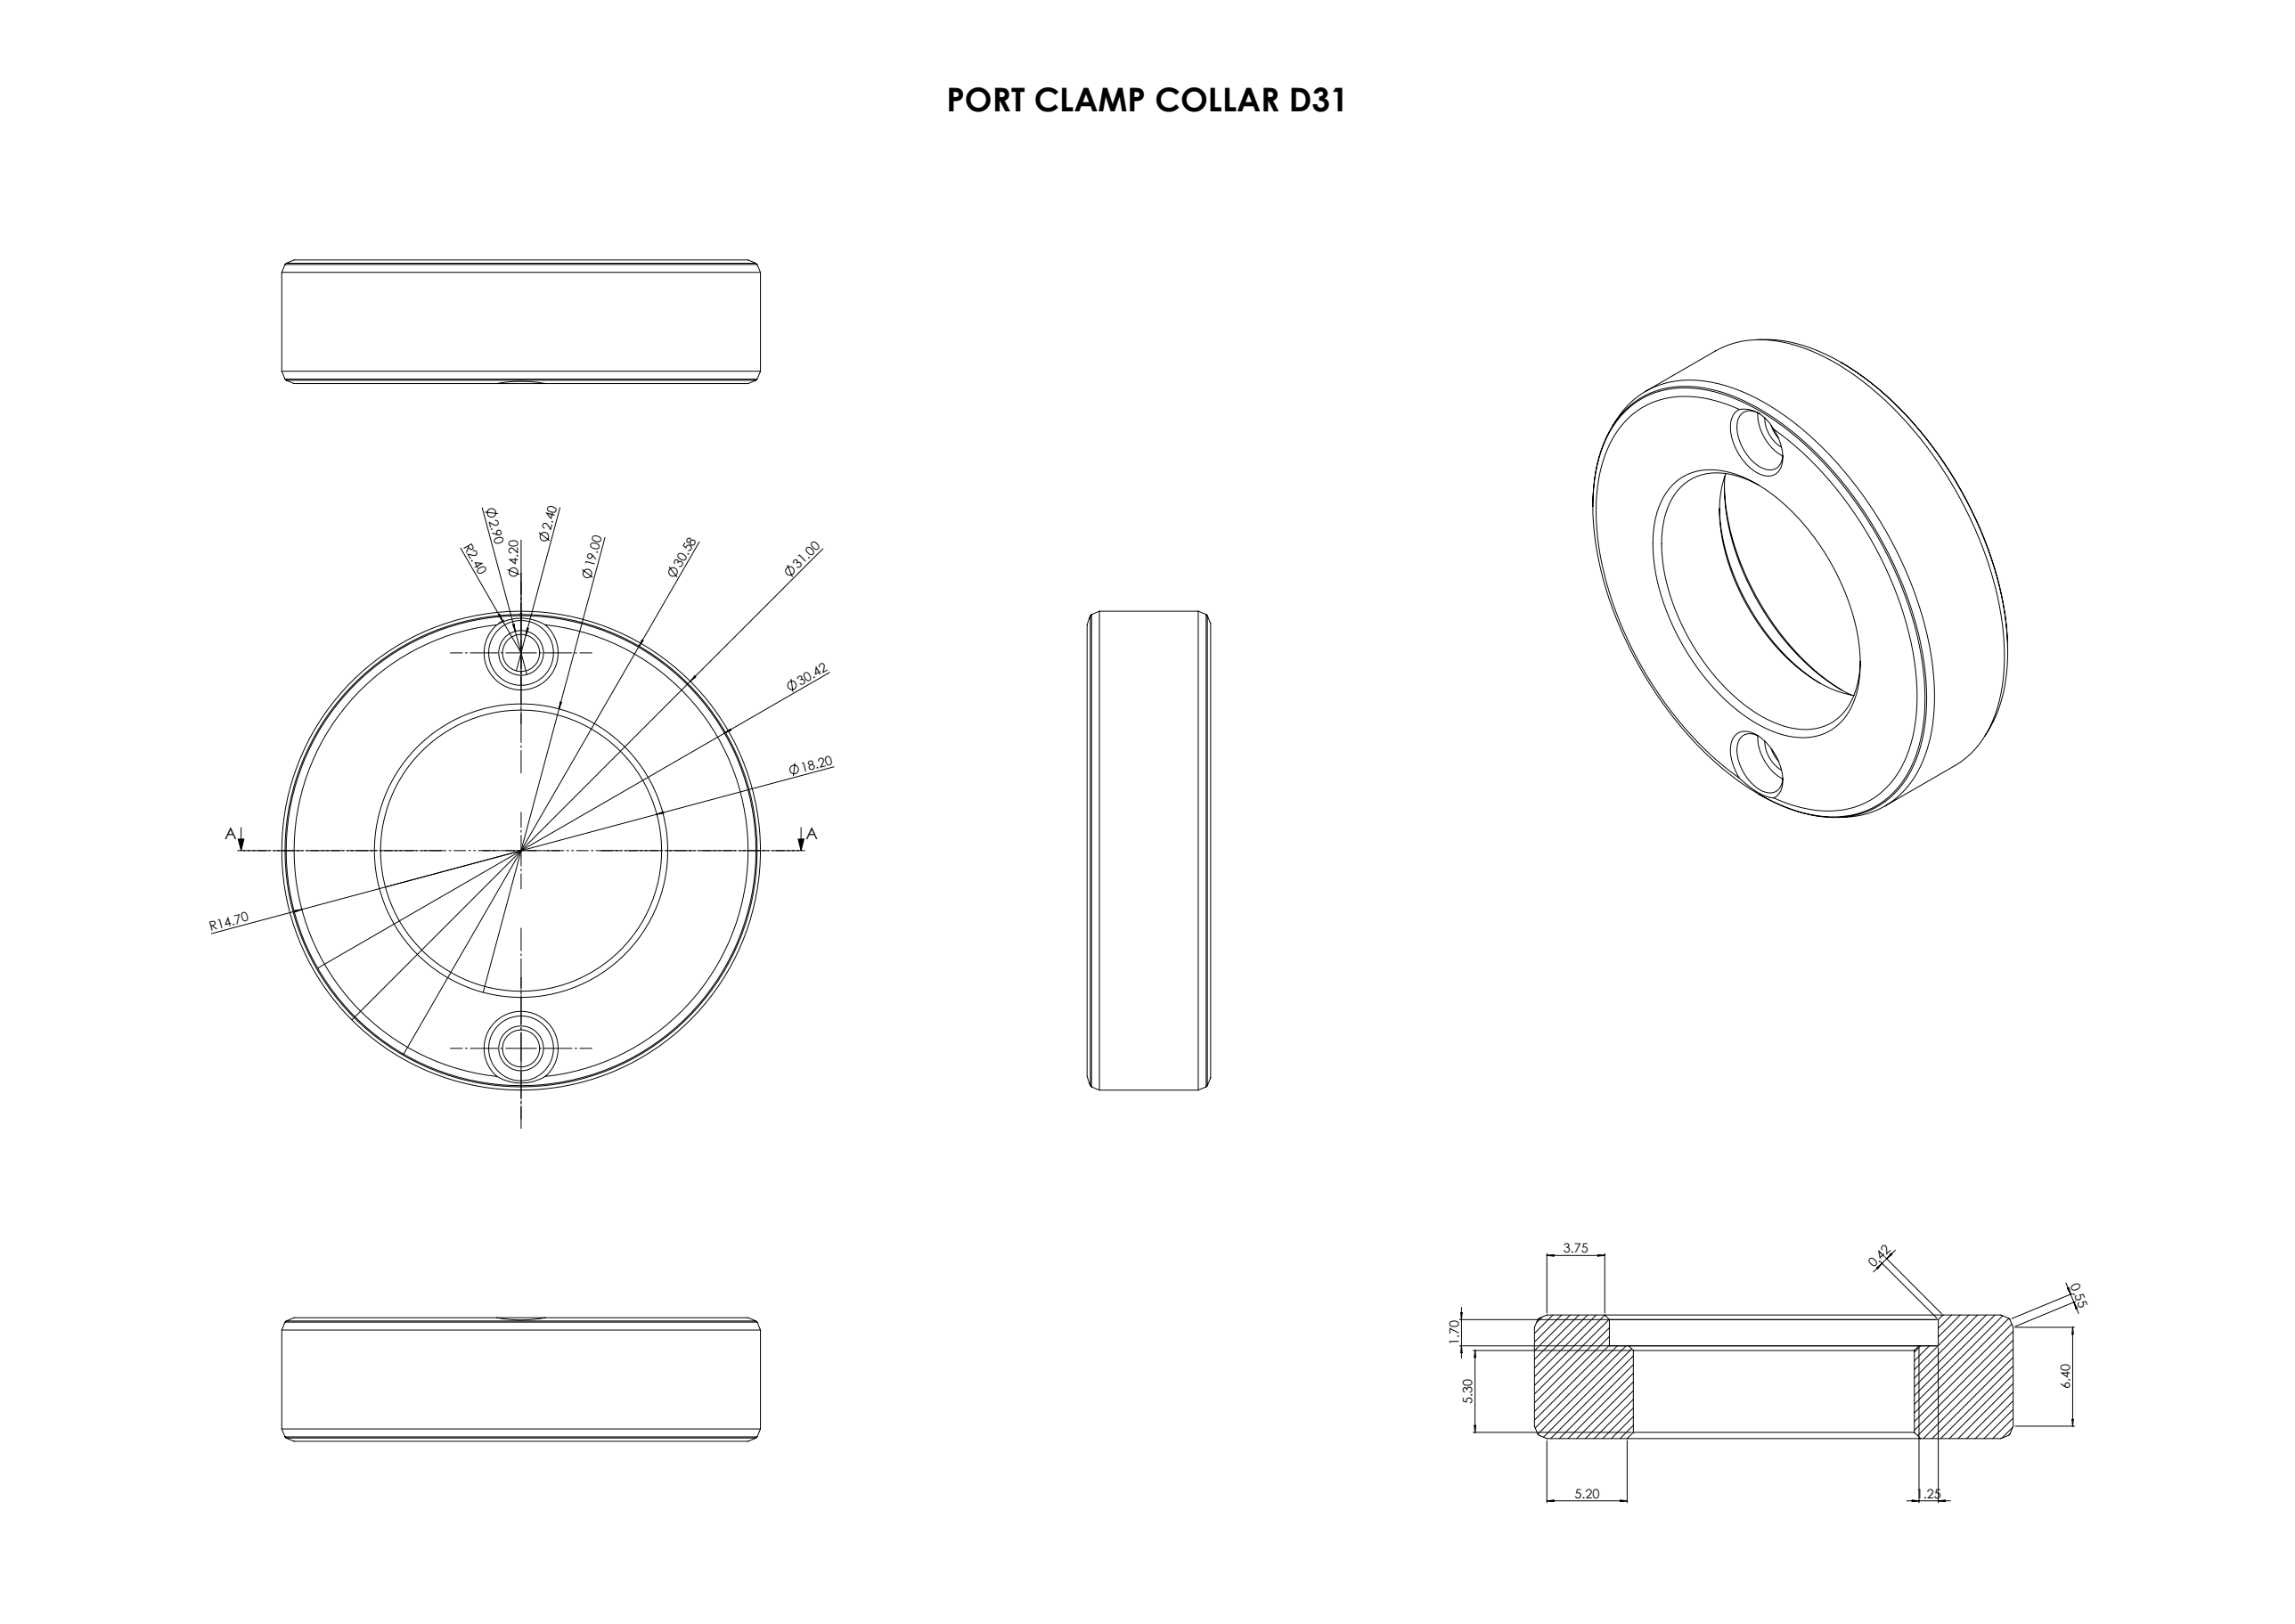
ISO-10303-21;
HEADER;
/* Generated by software containing ST-Developer
 * from STEP Tools, Inc. (www.steptools.com) 
 */

FILE_DESCRIPTION(
/* description */ (''),
/* implementation_level */ '2;1');

FILE_NAME(
/* name */ '05_Port_Clamp_Collar_D31.step',
/* time_stamp */ '2026-10-19T23:00:43-07:00',
/* author */ (''),
/* organization */ (''),
/* preprocessor_version */ 'ST-DEVELOPER v20.2',
/* originating_system */ 'Autodesk Translation Framework v15.15.0.0',
/* authorisation */ '');

FILE_SCHEMA (('AUTOMOTIVE_DESIGN { 1 0 10303 214 3 1 1 }'));
ENDSEC;

DATA;
#10=MECHANICAL_DESIGN_GEOMETRIC_PRESENTATION_REPRESENTATION('',(#1000),#55002);
#484=B_SPLINE_CURVE_WITH_KNOTS('',3,(#36025,#36026,#36027,#36028,#36029,
#36030,#36031,#36032,#36033,#36034),.UNSPECIFIED.,.F.,.F.,(4,2,2,2,4),(0.529829601296569,
0.55431923537737,0.690027699159176,0.825736162940983,0.850225797021783),
 .UNSPECIFIED.);
#485=B_SPLINE_CURVE_WITH_KNOTS('',3,(#36038,#36039,#36040,#36041,#36042,
#36043,#36044,#36045,#36046,#36047),.UNSPECIFIED.,.F.,.F.,(4,2,2,2,4),(0.529829601296585,
0.554319235377384,0.690027699159196,0.825736162941008,0.850225797021807),
 .UNSPECIFIED.);
#960=SHAPE_REPRESENTATION_RELATIONSHIP('SRR','None',#55108,#980);
#980=ADVANCED_BREP_SHAPE_REPRESENTATION('',(#1020),#54986);
#1000=STYLED_ITEM('',(#55379),#1020);
#1020=MANIFOLD_SOLID_BREP('Port Clamp Collar',#24533);
#1162=FACE_BOUND('',#4344,.T.);
#1163=FACE_BOUND('',#4345,.T.);
#1164=FACE_BOUND('',#4346,.T.);
#1165=FACE_BOUND('',#4357,.T.);
#1166=FACE_BOUND('',#4367,.T.);
#1167=FACE_BOUND('',#4372,.T.);
#1168=FACE_BOUND('',#4375,.T.);
#1418=PLANE('',#25686);
#1419=PLANE('',#25713);
#1420=PLANE('',#25738);
#1421=PLANE('',#25745);
#1422=PLANE('',#25748);
#2121=CYLINDRICAL_SURFACE('',#25690,1.065);
#2122=CYLINDRICAL_SURFACE('',#25699,1.55);
#2123=CYLINDRICAL_SURFACE('',#25710,0.91);
#2124=CYLINDRICAL_SURFACE('',#25723,0.21);
#2125=CYLINDRICAL_SURFACE('',#25730,0.21);
#2126=CYLINDRICAL_SURFACE('',#25734,0.12);
#2127=CYLINDRICAL_SURFACE('',#25741,0.12);
#2852=FACE_OUTER_BOUND('',#4342,.T.);
#2853=FACE_OUTER_BOUND('',#4343,.T.);
#2854=FACE_OUTER_BOUND('',#4347,.T.);
#2855=FACE_OUTER_BOUND('',#4348,.T.);
#2856=FACE_OUTER_BOUND('',#4349,.T.);
#2857=FACE_OUTER_BOUND('',#4350,.T.);
#2858=FACE_OUTER_BOUND('',#4351,.T.);
#2859=FACE_OUTER_BOUND('',#4352,.T.);
#2860=FACE_OUTER_BOUND('',#4353,.T.);
#2861=FACE_OUTER_BOUND('',#4354,.T.);
#2862=FACE_OUTER_BOUND('',#4355,.T.);
#2863=FACE_OUTER_BOUND('',#4356,.T.);
#2864=FACE_OUTER_BOUND('',#4358,.T.);
#2865=FACE_OUTER_BOUND('',#4359,.T.);
#2866=FACE_OUTER_BOUND('',#4360,.T.);
#2867=FACE_OUTER_BOUND('',#4361,.T.);
#2868=FACE_OUTER_BOUND('',#4362,.T.);
#2869=FACE_OUTER_BOUND('',#4363,.T.);
#2870=FACE_OUTER_BOUND('',#4364,.T.);
#2871=FACE_OUTER_BOUND('',#4365,.T.);
#2872=FACE_OUTER_BOUND('',#4366,.T.);
#2873=FACE_OUTER_BOUND('',#4368,.T.);
#2874=FACE_OUTER_BOUND('',#4369,.T.);
#2875=FACE_OUTER_BOUND('',#4370,.T.);
#2876=FACE_OUTER_BOUND('',#4371,.T.);
#2877=FACE_OUTER_BOUND('',#4373,.T.);
#2878=FACE_OUTER_BOUND('',#4374,.T.);
#4342=EDGE_LOOP('',(#17878,#17879,#17880,#17881,#17882));
#4343=EDGE_LOOP('',(#17883));
#4344=EDGE_LOOP('',(#17884));
#4345=EDGE_LOOP('',(#17885));
#4346=EDGE_LOOP('',(#17886));
#4347=EDGE_LOOP('',(#17887,#17888,#17889,#17890,#17891));
#4348=EDGE_LOOP('',(#17892,#17893,#17894,#17895));
#4349=EDGE_LOOP('',(#17896,#17897,#17898,#17899));
#4350=EDGE_LOOP('',(#17900,#17901,#17902,#17903,#17904));
#4351=EDGE_LOOP('',(#17905,#17906,#17907,#17908,#17909,#17910));
#4352=EDGE_LOOP('',(#17911,#17912,#17913,#17914,#17915));
#4353=EDGE_LOOP('',(#17916,#17917,#17918,#17919));
#4354=EDGE_LOOP('',(#17920,#17921,#17922,#17923,#17924));
#4355=EDGE_LOOP('',(#17925,#17926,#17927,#17928,#17929,#17930));
#4356=EDGE_LOOP('',(#17931));
#4357=EDGE_LOOP('',(#17932));
#4358=EDGE_LOOP('',(#17933,#17934,#17935,#17936,#17937,#17938,#17939,#17940));
#4359=EDGE_LOOP('',(#17941,#17942,#17943,#17944,#17945,#17946,#17947));
#4360=EDGE_LOOP('',(#17948,#17949,#17950,#17951,#17952));
#4361=EDGE_LOOP('',(#17953,#17954,#17955,#17956,#17957,#17958,#17959));
#4362=EDGE_LOOP('',(#17960,#17961,#17962,#17963,#17964));
#4363=EDGE_LOOP('',(#17965,#17966,#17967,#17968));
#4364=EDGE_LOOP('',(#17969,#17970,#17971,#17972));
#4365=EDGE_LOOP('',(#17973,#17974,#17975,#17976));
#4366=EDGE_LOOP('',(#17977));
#4367=EDGE_LOOP('',(#17978));
#4368=EDGE_LOOP('',(#17979,#17980,#17981,#17982));
#4369=EDGE_LOOP('',(#17983,#17984,#17985,#17986));
#4370=EDGE_LOOP('',(#17987,#17988,#17989,#17990));
#4371=EDGE_LOOP('',(#17991));
#4372=EDGE_LOOP('',(#17992));
#4373=EDGE_LOOP('',(#17993,#17994,#17995,#17996,#17997));
#4374=EDGE_LOOP('',(#17998,#17999,#18000,#18001,#18002,#18003,#18004));
#4375=EDGE_LOOP('',(#18005));
#5910=LINE('',#35961,#7731);
#5911=LINE('',#35975,#7732);
#5912=LINE('',#35979,#7733);
#5913=LINE('',#35983,#7734);
#5914=LINE('',#35986,#7735);
#5915=LINE('',#35995,#7736);
#5916=LINE('',#35999,#7737);
#5917=LINE('',#36003,#7738);
#5918=LINE('',#36008,#7739);
#5919=LINE('',#36017,#7740);
#5920=LINE('',#36021,#7741);
#5921=LINE('',#36053,#7742);
#5922=LINE('',#36061,#7743);
#5923=LINE('',#36066,#7744);
#5924=LINE('',#36074,#7745);
#5925=LINE('',#36077,#7746);
#5926=LINE('',#36081,#7747);
#5927=LINE('',#36085,#7748);
#5928=LINE('',#36090,#7749);
#5929=LINE('',#36094,#7750);
#5930=LINE('',#36098,#7751);
#5931=LINE('',#36103,#7752);
#7731=VECTOR('',#29554,1.08);
#7732=VECTOR('',#29571,1.065);
#7733=VECTOR('',#29576,1.4956066017178);
#7734=VECTOR('',#29581,1.525);
#7735=VECTOR('',#29584,1.5393933982822);
#7736=VECTOR('',#29595,1.55);
#7737=VECTOR('',#29600,1.5393933982822);
#7738=VECTOR('',#29605,1.525);
#7739=VECTOR('',#29610,0.925);
#7740=VECTOR('',#29621,0.91);
#7741=VECTOR('',#29626,1.4956066017178);
#7742=VECTOR('',#29637,0.225);
#7743=VECTOR('',#29648,0.21);
#7744=VECTOR('',#29653,0.225);
#7745=VECTOR('',#29664,0.21);
#7746=VECTOR('',#29667,0.1325);
#7747=VECTOR('',#29672,0.12);
#7748=VECTOR('',#29677,0.1325);
#7749=VECTOR('',#29684,0.1325);
#7750=VECTOR('',#29689,0.12);
#7751=VECTOR('',#29694,0.1325);
#7752=VECTOR('',#29701,0.93);
#9488=CIRCLE('',#25683,1.095);
#9489=CIRCLE('',#25684,1.065);
#9490=CIRCLE('',#25685,1.065);
#9491=CIRCLE('',#25687,1.47);
#9492=CIRCLE('',#25688,0.128333333333334);
#9493=CIRCLE('',#25689,0.128333333333334);
#9494=CIRCLE('',#25691,1.065);
#9495=CIRCLE('',#25693,1.5212132034356);
#9496=CIRCLE('',#25695,1.5287867965644);
#9497=CIRCLE('',#25697,1.55);
#9498=CIRCLE('',#25698,1.55);
#9499=CIRCLE('',#25700,1.55);
#9500=CIRCLE('',#25701,1.55);
#9501=CIRCLE('',#25703,1.5287867965644);
#9502=CIRCLE('',#25705,1.5212132034356);
#9503=CIRCLE('',#25707,0.94);
#9504=CIRCLE('',#25708,0.91);
#9505=CIRCLE('',#25709,0.91);
#9506=CIRCLE('',#25711,0.91);
#9507=CIRCLE('',#25712,0.91);
#9508=CIRCLE('',#25715,1.47);
#9509=CIRCLE('',#25716,1.47);
#9510=CIRCLE('',#25717,1.47);
#9511=CIRCLE('',#25719,0.24);
#9512=CIRCLE('',#25720,0.21);
#9513=CIRCLE('',#25721,0.21);
#9514=CIRCLE('',#25722,0.24);
#9515=CIRCLE('',#25724,0.21);
#9516=CIRCLE('',#25726,0.24);
#9517=CIRCLE('',#25727,0.21);
#9518=CIRCLE('',#25728,0.21);
#9519=CIRCLE('',#25729,0.24);
#9520=CIRCLE('',#25731,0.21);
#9521=CIRCLE('',#25733,0.12);
#9522=CIRCLE('',#25735,0.12);
#9523=CIRCLE('',#25737,0.145);
#9524=CIRCLE('',#25740,0.12);
#9525=CIRCLE('',#25742,0.12);
#9526=CIRCLE('',#25744,0.145);
#9527=CIRCLE('',#25747,0.95);
#10672=VERTEX_POINT('',#35958);
#10673=VERTEX_POINT('',#35960);
#10674=VERTEX_POINT('',#35962);
#10675=VERTEX_POINT('',#35966);
#10676=VERTEX_POINT('',#35968);
#10677=VERTEX_POINT('',#35970);
#10678=VERTEX_POINT('',#35973);
#10679=VERTEX_POINT('',#35977);
#10680=VERTEX_POINT('',#35981);
#10681=VERTEX_POINT('',#35985);
#10682=VERTEX_POINT('',#35987);
#10683=VERTEX_POINT('',#35991);
#10684=VERTEX_POINT('',#35992);
#10685=VERTEX_POINT('',#35997);
#10686=VERTEX_POINT('',#36001);
#10687=VERTEX_POINT('',#36005);
#10688=VERTEX_POINT('',#36007);
#10689=VERTEX_POINT('',#36009);
#10690=VERTEX_POINT('',#36013);
#10691=VERTEX_POINT('',#36014);
#10692=VERTEX_POINT('',#36020);
#10693=VERTEX_POINT('',#36022);
#10694=VERTEX_POINT('',#36024);
#10695=VERTEX_POINT('',#36035);
#10696=VERTEX_POINT('',#36037);
#10697=VERTEX_POINT('',#36050);
#10698=VERTEX_POINT('',#36052);
#10699=VERTEX_POINT('',#36054);
#10700=VERTEX_POINT('',#36059);
#10701=VERTEX_POINT('',#36063);
#10702=VERTEX_POINT('',#36065);
#10703=VERTEX_POINT('',#36067);
#10704=VERTEX_POINT('',#36072);
#10705=VERTEX_POINT('',#36076);
#10706=VERTEX_POINT('',#36080);
#10707=VERTEX_POINT('',#36084);
#10708=VERTEX_POINT('',#36089);
#10709=VERTEX_POINT('',#36093);
#10710=VERTEX_POINT('',#36097);
#10711=VERTEX_POINT('',#36102);
#13347=EDGE_CURVE('',#10672,#10672,#9488,.T.);
#13348=EDGE_CURVE('',#10672,#10673,#5910,.T.);
#13349=EDGE_CURVE('',#10673,#10674,#9489,.T.);
#13350=EDGE_CURVE('',#10674,#10673,#9490,.T.);
#13351=EDGE_CURVE('',#10675,#10675,#9491,.T.);
#13352=EDGE_CURVE('',#10676,#10676,#9492,.T.);
#13353=EDGE_CURVE('',#10677,#10677,#9493,.T.);
#13354=EDGE_CURVE('',#10678,#10678,#9494,.T.);
#13355=EDGE_CURVE('',#10678,#10674,#5911,.T.);
#13356=EDGE_CURVE('',#10679,#10679,#9495,.T.);
#13357=EDGE_CURVE('',#10679,#10675,#5912,.T.);
#13358=EDGE_CURVE('',#10680,#10680,#9496,.T.);
#13359=EDGE_CURVE('',#10680,#10679,#5913,.T.);
#13360=EDGE_CURVE('',#10680,#10681,#5914,.T.);
#13361=EDGE_CURVE('',#10681,#10682,#9497,.T.);
#13362=EDGE_CURVE('',#10682,#10681,#9498,.T.);
#13363=EDGE_CURVE('',#10683,#10684,#9499,.T.);
#13364=EDGE_CURVE('',#10684,#10683,#9500,.T.);
#13365=EDGE_CURVE('',#10684,#10682,#5915,.T.);
#13366=EDGE_CURVE('',#10685,#10685,#9501,.T.);
#13367=EDGE_CURVE('',#10685,#10683,#5916,.T.);
#13368=EDGE_CURVE('',#10686,#10686,#9502,.T.);
#13369=EDGE_CURVE('',#10686,#10685,#5917,.T.);
#13370=EDGE_CURVE('',#10687,#10687,#9503,.T.);
#13371=EDGE_CURVE('',#10687,#10688,#5918,.T.);
#13372=EDGE_CURVE('',#10688,#10689,#9504,.T.);
#13373=EDGE_CURVE('',#10689,#10688,#9505,.T.);
#13374=EDGE_CURVE('',#10690,#10691,#9506,.T.);
#13375=EDGE_CURVE('',#10691,#10690,#9507,.T.);
#13376=EDGE_CURVE('',#10691,#10689,#5919,.T.);
#13377=EDGE_CURVE('',#10686,#10692,#5920,.T.);
#13378=EDGE_CURVE('',#10692,#10693,#9508,.T.);
#13379=EDGE_CURVE('',#10694,#10693,#484,.T.);
#13380=EDGE_CURVE('',#10694,#10695,#9509,.T.);
#13381=EDGE_CURVE('',#10696,#10695,#485,.T.);
#13382=EDGE_CURVE('',#10696,#10692,#9510,.T.);
#13383=EDGE_CURVE('',#10695,#10697,#9511,.T.);
#13384=EDGE_CURVE('',#10697,#10698,#5921,.T.);
#13385=EDGE_CURVE('',#10698,#10699,#9512,.T.);
#13386=EDGE_CURVE('',#10699,#10698,#9513,.T.);
#13387=EDGE_CURVE('',#10697,#10696,#9514,.T.);
#13388=EDGE_CURVE('',#10700,#10700,#9515,.T.);
#13389=EDGE_CURVE('',#10700,#10699,#5922,.T.);
#13390=EDGE_CURVE('',#10693,#10701,#9516,.T.);
#13391=EDGE_CURVE('',#10701,#10702,#5923,.T.);
#13392=EDGE_CURVE('',#10702,#10703,#9517,.T.);
#13393=EDGE_CURVE('',#10703,#10702,#9518,.T.);
#13394=EDGE_CURVE('',#10701,#10694,#9519,.T.);
#13395=EDGE_CURVE('',#10704,#10704,#9520,.T.);
#13396=EDGE_CURVE('',#10704,#10703,#5924,.T.);
#13397=EDGE_CURVE('',#10676,#10705,#5925,.T.);
#13398=EDGE_CURVE('',#10705,#10705,#9521,.T.);
#13399=EDGE_CURVE('',#10705,#10706,#5926,.T.);
#13400=EDGE_CURVE('',#10706,#10706,#9522,.T.);
#13401=EDGE_CURVE('',#10706,#10707,#5927,.T.);
#13402=EDGE_CURVE('',#10707,#10707,#9523,.T.);
#13403=EDGE_CURVE('',#10677,#10708,#5928,.T.);
#13404=EDGE_CURVE('',#10708,#10708,#9524,.T.);
#13405=EDGE_CURVE('',#10708,#10709,#5929,.T.);
#13406=EDGE_CURVE('',#10709,#10709,#9525,.T.);
#13407=EDGE_CURVE('',#10709,#10710,#5930,.T.);
#13408=EDGE_CURVE('',#10710,#10710,#9526,.T.);
#13409=EDGE_CURVE('',#10690,#10711,#5931,.T.);
#13410=EDGE_CURVE('',#10711,#10711,#9527,.T.);
#17878=ORIENTED_EDGE('',*,*,#13347,.T.);
#17879=ORIENTED_EDGE('',*,*,#13348,.T.);
#17880=ORIENTED_EDGE('',*,*,#13349,.T.);
#17881=ORIENTED_EDGE('',*,*,#13350,.T.);
#17882=ORIENTED_EDGE('',*,*,#13348,.F.);
#17883=ORIENTED_EDGE('',*,*,#13351,.F.);
#17884=ORIENTED_EDGE('',*,*,#13352,.T.);
#17885=ORIENTED_EDGE('',*,*,#13353,.T.);
#17886=ORIENTED_EDGE('',*,*,#13347,.F.);
#17887=ORIENTED_EDGE('',*,*,#13354,.T.);
#17888=ORIENTED_EDGE('',*,*,#13355,.T.);
#17889=ORIENTED_EDGE('',*,*,#13349,.F.);
#17890=ORIENTED_EDGE('',*,*,#13350,.F.);
#17891=ORIENTED_EDGE('',*,*,#13355,.F.);
#17892=ORIENTED_EDGE('',*,*,#13356,.T.);
#17893=ORIENTED_EDGE('',*,*,#13357,.T.);
#17894=ORIENTED_EDGE('',*,*,#13351,.T.);
#17895=ORIENTED_EDGE('',*,*,#13357,.F.);
#17896=ORIENTED_EDGE('',*,*,#13358,.F.);
#17897=ORIENTED_EDGE('',*,*,#13359,.T.);
#17898=ORIENTED_EDGE('',*,*,#13356,.F.);
#17899=ORIENTED_EDGE('',*,*,#13359,.F.);
#17900=ORIENTED_EDGE('',*,*,#13358,.T.);
#17901=ORIENTED_EDGE('',*,*,#13360,.T.);
#17902=ORIENTED_EDGE('',*,*,#13361,.T.);
#17903=ORIENTED_EDGE('',*,*,#13362,.T.);
#17904=ORIENTED_EDGE('',*,*,#13360,.F.);
#17905=ORIENTED_EDGE('',*,*,#13363,.F.);
#17906=ORIENTED_EDGE('',*,*,#13364,.F.);
#17907=ORIENTED_EDGE('',*,*,#13365,.T.);
#17908=ORIENTED_EDGE('',*,*,#13361,.F.);
#17909=ORIENTED_EDGE('',*,*,#13362,.F.);
#17910=ORIENTED_EDGE('',*,*,#13365,.F.);
#17911=ORIENTED_EDGE('',*,*,#13366,.T.);
#17912=ORIENTED_EDGE('',*,*,#13367,.T.);
#17913=ORIENTED_EDGE('',*,*,#13363,.T.);
#17914=ORIENTED_EDGE('',*,*,#13364,.T.);
#17915=ORIENTED_EDGE('',*,*,#13367,.F.);
#17916=ORIENTED_EDGE('',*,*,#13368,.F.);
#17917=ORIENTED_EDGE('',*,*,#13369,.T.);
#17918=ORIENTED_EDGE('',*,*,#13366,.F.);
#17919=ORIENTED_EDGE('',*,*,#13369,.F.);
#17920=ORIENTED_EDGE('',*,*,#13370,.T.);
#17921=ORIENTED_EDGE('',*,*,#13371,.T.);
#17922=ORIENTED_EDGE('',*,*,#13372,.T.);
#17923=ORIENTED_EDGE('',*,*,#13373,.T.);
#17924=ORIENTED_EDGE('',*,*,#13371,.F.);
#17925=ORIENTED_EDGE('',*,*,#13374,.F.);
#17926=ORIENTED_EDGE('',*,*,#13375,.F.);
#17927=ORIENTED_EDGE('',*,*,#13376,.T.);
#17928=ORIENTED_EDGE('',*,*,#13372,.F.);
#17929=ORIENTED_EDGE('',*,*,#13373,.F.);
#17930=ORIENTED_EDGE('',*,*,#13376,.F.);
#17931=ORIENTED_EDGE('',*,*,#13354,.F.);
#17932=ORIENTED_EDGE('',*,*,#13370,.F.);
#17933=ORIENTED_EDGE('',*,*,#13368,.T.);
#17934=ORIENTED_EDGE('',*,*,#13377,.T.);
#17935=ORIENTED_EDGE('',*,*,#13378,.T.);
#17936=ORIENTED_EDGE('',*,*,#13379,.F.);
#17937=ORIENTED_EDGE('',*,*,#13380,.T.);
#17938=ORIENTED_EDGE('',*,*,#13381,.F.);
#17939=ORIENTED_EDGE('',*,*,#13382,.T.);
#17940=ORIENTED_EDGE('',*,*,#13377,.F.);
#17941=ORIENTED_EDGE('',*,*,#13381,.T.);
#17942=ORIENTED_EDGE('',*,*,#13383,.T.);
#17943=ORIENTED_EDGE('',*,*,#13384,.T.);
#17944=ORIENTED_EDGE('',*,*,#13385,.T.);
#17945=ORIENTED_EDGE('',*,*,#13386,.T.);
#17946=ORIENTED_EDGE('',*,*,#13384,.F.);
#17947=ORIENTED_EDGE('',*,*,#13387,.T.);
#17948=ORIENTED_EDGE('',*,*,#13388,.F.);
#17949=ORIENTED_EDGE('',*,*,#13389,.T.);
#17950=ORIENTED_EDGE('',*,*,#13385,.F.);
#17951=ORIENTED_EDGE('',*,*,#13386,.F.);
#17952=ORIENTED_EDGE('',*,*,#13389,.F.);
#17953=ORIENTED_EDGE('',*,*,#13379,.T.);
#17954=ORIENTED_EDGE('',*,*,#13390,.T.);
#17955=ORIENTED_EDGE('',*,*,#13391,.T.);
#17956=ORIENTED_EDGE('',*,*,#13392,.T.);
#17957=ORIENTED_EDGE('',*,*,#13393,.T.);
#17958=ORIENTED_EDGE('',*,*,#13391,.F.);
#17959=ORIENTED_EDGE('',*,*,#13394,.T.);
#17960=ORIENTED_EDGE('',*,*,#13395,.F.);
#17961=ORIENTED_EDGE('',*,*,#13396,.T.);
#17962=ORIENTED_EDGE('',*,*,#13392,.F.);
#17963=ORIENTED_EDGE('',*,*,#13393,.F.);
#17964=ORIENTED_EDGE('',*,*,#13396,.F.);
#17965=ORIENTED_EDGE('',*,*,#13352,.F.);
#17966=ORIENTED_EDGE('',*,*,#13397,.T.);
#17967=ORIENTED_EDGE('',*,*,#13398,.T.);
#17968=ORIENTED_EDGE('',*,*,#13397,.F.);
#17969=ORIENTED_EDGE('',*,*,#13398,.F.);
#17970=ORIENTED_EDGE('',*,*,#13399,.T.);
#17971=ORIENTED_EDGE('',*,*,#13400,.T.);
#17972=ORIENTED_EDGE('',*,*,#13399,.F.);
#17973=ORIENTED_EDGE('',*,*,#13400,.F.);
#17974=ORIENTED_EDGE('',*,*,#13401,.T.);
#17975=ORIENTED_EDGE('',*,*,#13402,.T.);
#17976=ORIENTED_EDGE('',*,*,#13401,.F.);
#17977=ORIENTED_EDGE('',*,*,#13395,.T.);
#17978=ORIENTED_EDGE('',*,*,#13402,.F.);
#17979=ORIENTED_EDGE('',*,*,#13353,.F.);
#17980=ORIENTED_EDGE('',*,*,#13403,.T.);
#17981=ORIENTED_EDGE('',*,*,#13404,.T.);
#17982=ORIENTED_EDGE('',*,*,#13403,.F.);
#17983=ORIENTED_EDGE('',*,*,#13404,.F.);
#17984=ORIENTED_EDGE('',*,*,#13405,.T.);
#17985=ORIENTED_EDGE('',*,*,#13406,.T.);
#17986=ORIENTED_EDGE('',*,*,#13405,.F.);
#17987=ORIENTED_EDGE('',*,*,#13406,.F.);
#17988=ORIENTED_EDGE('',*,*,#13407,.T.);
#17989=ORIENTED_EDGE('',*,*,#13408,.T.);
#17990=ORIENTED_EDGE('',*,*,#13407,.F.);
#17991=ORIENTED_EDGE('',*,*,#13388,.T.);
#17992=ORIENTED_EDGE('',*,*,#13408,.F.);
#17993=ORIENTED_EDGE('',*,*,#13374,.T.);
#17994=ORIENTED_EDGE('',*,*,#13375,.T.);
#17995=ORIENTED_EDGE('',*,*,#13409,.T.);
#17996=ORIENTED_EDGE('',*,*,#13410,.T.);
#17997=ORIENTED_EDGE('',*,*,#13409,.F.);
#17998=ORIENTED_EDGE('',*,*,#13382,.F.);
#17999=ORIENTED_EDGE('',*,*,#13387,.F.);
#18000=ORIENTED_EDGE('',*,*,#13383,.F.);
#18001=ORIENTED_EDGE('',*,*,#13380,.F.);
#18002=ORIENTED_EDGE('',*,*,#13394,.F.);
#18003=ORIENTED_EDGE('',*,*,#13390,.F.);
#18004=ORIENTED_EDGE('',*,*,#13378,.F.);
#18005=ORIENTED_EDGE('',*,*,#13410,.F.);
#23083=CONICAL_SURFACE('',#25682,1.08,0.785398163397459);
#23084=CONICAL_SURFACE('',#25692,1.4956066017178,1.17809724509617);
#23085=CONICAL_SURFACE('',#25694,1.525,0.785398163397442);
#23086=CONICAL_SURFACE('',#25696,1.5393933982822,0.392699081698728);
#23087=CONICAL_SURFACE('',#25702,1.5393933982822,0.392699081698728);
#23088=CONICAL_SURFACE('',#25704,1.525,0.785398163397442);
#23089=CONICAL_SURFACE('',#25706,0.925,0.785398163397459);
#23090=CONICAL_SURFACE('',#25714,1.4956066017178,1.17809724509617);
#23091=CONICAL_SURFACE('',#25718,0.225,0.785398163397459);
#23092=CONICAL_SURFACE('',#25725,0.225,0.785398163397459);
#23093=CONICAL_SURFACE('',#25732,0.1325,0.321750554396645);
#23094=CONICAL_SURFACE('',#25736,0.1325,0.785398163397441);
#23095=CONICAL_SURFACE('',#25739,0.1325,0.321750554396645);
#23096=CONICAL_SURFACE('',#25743,0.1325,0.785398163397441);
#23097=CONICAL_SURFACE('',#25746,0.93,0.785398163397459);
#23605=ADVANCED_FACE('',(#2852),#23083,.F.);
#23606=ADVANCED_FACE('',(#2853,#1162,#1163,#1164),#1418,.T.);
#23607=ADVANCED_FACE('',(#2854),#2121,.F.);
#23608=ADVANCED_FACE('',(#2855),#23084,.T.);
#23609=ADVANCED_FACE('',(#2856),#23085,.T.);
#23610=ADVANCED_FACE('',(#2857),#23086,.T.);
#23611=ADVANCED_FACE('',(#2858),#2122,.T.);
#23612=ADVANCED_FACE('',(#2859),#23087,.T.);
#23613=ADVANCED_FACE('',(#2860),#23088,.T.);
#23614=ADVANCED_FACE('',(#2861),#23089,.F.);
#23615=ADVANCED_FACE('',(#2862),#2123,.F.);
#23616=ADVANCED_FACE('',(#2863,#1165),#1419,.T.);
#23617=ADVANCED_FACE('',(#2864),#23090,.T.);
#23618=ADVANCED_FACE('',(#2865),#23091,.F.);
#23619=ADVANCED_FACE('',(#2866),#2124,.F.);
#23620=ADVANCED_FACE('',(#2867),#23092,.F.);
#23621=ADVANCED_FACE('',(#2868),#2125,.F.);
#23622=ADVANCED_FACE('',(#2869),#23093,.F.);
#23623=ADVANCED_FACE('',(#2870),#2126,.F.);
#23624=ADVANCED_FACE('',(#2871),#23094,.F.);
#23625=ADVANCED_FACE('',(#2872,#1166),#1420,.F.);
#23626=ADVANCED_FACE('',(#2873),#23095,.F.);
#23627=ADVANCED_FACE('',(#2874),#2127,.F.);
#23628=ADVANCED_FACE('',(#2875),#23096,.F.);
#23629=ADVANCED_FACE('',(#2876,#1167),#1421,.F.);
#23630=ADVANCED_FACE('',(#2877),#23097,.F.);
#23631=ADVANCED_FACE('',(#2878,#1168),#1422,.T.);
#24533=CLOSED_SHELL('',(#23605,#23606,#23607,#23608,#23609,#23610,#23611,
#23612,#23613,#23614,#23615,#23616,#23617,#23618,#23619,#23620,#23621,#23622,
#23623,#23624,#23625,#23626,#23627,#23628,#23629,#23630,#23631));
#25681=AXIS2_PLACEMENT_3D('',#35956,#29548,#29549);
#25682=AXIS2_PLACEMENT_3D('',#35957,#29550,#29551);
#25683=AXIS2_PLACEMENT_3D('',#35959,#29552,#29553);
#25684=AXIS2_PLACEMENT_3D('',#35963,#29555,#29556);
#25685=AXIS2_PLACEMENT_3D('',#35964,#29557,#29558);
#25686=AXIS2_PLACEMENT_3D('',#35965,#29559,#29560);
#25687=AXIS2_PLACEMENT_3D('',#35967,#29561,#29562);
#25688=AXIS2_PLACEMENT_3D('',#35969,#29563,#29564);
#25689=AXIS2_PLACEMENT_3D('',#35971,#29565,#29566);
#25690=AXIS2_PLACEMENT_3D('',#35972,#29567,#29568);
#25691=AXIS2_PLACEMENT_3D('',#35974,#29569,#29570);
#25692=AXIS2_PLACEMENT_3D('',#35976,#29572,#29573);
#25693=AXIS2_PLACEMENT_3D('',#35978,#29574,#29575);
#25694=AXIS2_PLACEMENT_3D('',#35980,#29577,#29578);
#25695=AXIS2_PLACEMENT_3D('',#35982,#29579,#29580);
#25696=AXIS2_PLACEMENT_3D('',#35984,#29582,#29583);
#25697=AXIS2_PLACEMENT_3D('',#35988,#29585,#29586);
#25698=AXIS2_PLACEMENT_3D('',#35989,#29587,#29588);
#25699=AXIS2_PLACEMENT_3D('',#35990,#29589,#29590);
#25700=AXIS2_PLACEMENT_3D('',#35993,#29591,#29592);
#25701=AXIS2_PLACEMENT_3D('',#35994,#29593,#29594);
#25702=AXIS2_PLACEMENT_3D('',#35996,#29596,#29597);
#25703=AXIS2_PLACEMENT_3D('',#35998,#29598,#29599);
#25704=AXIS2_PLACEMENT_3D('',#36000,#29601,#29602);
#25705=AXIS2_PLACEMENT_3D('',#36002,#29603,#29604);
#25706=AXIS2_PLACEMENT_3D('',#36004,#29606,#29607);
#25707=AXIS2_PLACEMENT_3D('',#36006,#29608,#29609);
#25708=AXIS2_PLACEMENT_3D('',#36010,#29611,#29612);
#25709=AXIS2_PLACEMENT_3D('',#36011,#29613,#29614);
#25710=AXIS2_PLACEMENT_3D('',#36012,#29615,#29616);
#25711=AXIS2_PLACEMENT_3D('',#36015,#29617,#29618);
#25712=AXIS2_PLACEMENT_3D('',#36016,#29619,#29620);
#25713=AXIS2_PLACEMENT_3D('',#36018,#29622,#29623);
#25714=AXIS2_PLACEMENT_3D('',#36019,#29624,#29625);
#25715=AXIS2_PLACEMENT_3D('',#36023,#29627,#29628);
#25716=AXIS2_PLACEMENT_3D('',#36036,#29629,#29630);
#25717=AXIS2_PLACEMENT_3D('',#36048,#29631,#29632);
#25718=AXIS2_PLACEMENT_3D('',#36049,#29633,#29634);
#25719=AXIS2_PLACEMENT_3D('',#36051,#29635,#29636);
#25720=AXIS2_PLACEMENT_3D('',#36055,#29638,#29639);
#25721=AXIS2_PLACEMENT_3D('',#36056,#29640,#29641);
#25722=AXIS2_PLACEMENT_3D('',#36057,#29642,#29643);
#25723=AXIS2_PLACEMENT_3D('',#36058,#29644,#29645);
#25724=AXIS2_PLACEMENT_3D('',#36060,#29646,#29647);
#25725=AXIS2_PLACEMENT_3D('',#36062,#29649,#29650);
#25726=AXIS2_PLACEMENT_3D('',#36064,#29651,#29652);
#25727=AXIS2_PLACEMENT_3D('',#36068,#29654,#29655);
#25728=AXIS2_PLACEMENT_3D('',#36069,#29656,#29657);
#25729=AXIS2_PLACEMENT_3D('',#36070,#29658,#29659);
#25730=AXIS2_PLACEMENT_3D('',#36071,#29660,#29661);
#25731=AXIS2_PLACEMENT_3D('',#36073,#29662,#29663);
#25732=AXIS2_PLACEMENT_3D('',#36075,#29665,#29666);
#25733=AXIS2_PLACEMENT_3D('',#36078,#29668,#29669);
#25734=AXIS2_PLACEMENT_3D('',#36079,#29670,#29671);
#25735=AXIS2_PLACEMENT_3D('',#36082,#29673,#29674);
#25736=AXIS2_PLACEMENT_3D('',#36083,#29675,#29676);
#25737=AXIS2_PLACEMENT_3D('',#36086,#29678,#29679);
#25738=AXIS2_PLACEMENT_3D('',#36087,#29680,#29681);
#25739=AXIS2_PLACEMENT_3D('',#36088,#29682,#29683);
#25740=AXIS2_PLACEMENT_3D('',#36091,#29685,#29686);
#25741=AXIS2_PLACEMENT_3D('',#36092,#29687,#29688);
#25742=AXIS2_PLACEMENT_3D('',#36095,#29690,#29691);
#25743=AXIS2_PLACEMENT_3D('',#36096,#29692,#29693);
#25744=AXIS2_PLACEMENT_3D('',#36099,#29695,#29696);
#25745=AXIS2_PLACEMENT_3D('',#36100,#29697,#29698);
#25746=AXIS2_PLACEMENT_3D('',#36101,#29699,#29700);
#25747=AXIS2_PLACEMENT_3D('',#36104,#29702,#29703);
#25748=AXIS2_PLACEMENT_3D('',#36105,#29704,#29705);
#29548=DIRECTION('axis',(0.,0.,1.));
#29549=DIRECTION('refdir',(1.,0.,0.));
#29550=DIRECTION('center_axis',(0.,0.,-1.));
#29551=DIRECTION('ref_axis',(-1.,0.,0.));
#29552=DIRECTION('center_axis',(0.,0.,-1.));
#29553=DIRECTION('ref_axis',(-1.,0.,0.));
#29554=DIRECTION('',(-0.707106781186555,8.65956056235503E-17,0.70710678118654));
#29555=DIRECTION('center_axis',(0.,0.,1.));
#29556=DIRECTION('ref_axis',(-1.,0.,0.));
#29557=DIRECTION('center_axis',(0.,0.,1.));
#29558=DIRECTION('ref_axis',(-1.,0.,0.));
#29559=DIRECTION('center_axis',(0.,0.,-1.));
#29560=DIRECTION('ref_axis',(-1.,0.,0.));
#29561=DIRECTION('center_axis',(0.,0.,1.));
#29562=DIRECTION('ref_axis',(-1.,0.,0.));
#29563=DIRECTION('center_axis',(0.,0.,1.));
#29564=DIRECTION('ref_axis',(1.,0.,0.));
#29565=DIRECTION('center_axis',(0.,0.,1.));
#29566=DIRECTION('ref_axis',(1.,0.,0.));
#29567=DIRECTION('center_axis',(0.,0.,1.));
#29568=DIRECTION('ref_axis',(1.,0.,0.));
#29569=DIRECTION('center_axis',(0.,0.,1.));
#29570=DIRECTION('ref_axis',(1.,0.,0.));
#29571=DIRECTION('',(0.,0.,-1.));
#29572=DIRECTION('center_axis',(0.,4.39101262113477E-15,1.));
#29573=DIRECTION('ref_axis',(-1.,-3.11403559978336E-17,0.));
#29574=DIRECTION('center_axis',(0.,0.,-1.));
#29575=DIRECTION('ref_axis',(-1.,-6.12323399573677E-17,0.));
#29576=DIRECTION('',(-0.923879532511284,-1.8222803301846E-15,-0.382683432365097));
#29577=DIRECTION('center_axis',(0.,0.,1.));
#29578=DIRECTION('ref_axis',(-1.,0.,0.));
#29579=DIRECTION('center_axis',(0.,0.,1.));
#29580=DIRECTION('ref_axis',(-1.,-6.12323399573677E-17,0.));
#29581=DIRECTION('',(-0.707106781186543,-8.65956056235487E-17,-0.707106781186552));
#29582=DIRECTION('center_axis',(0.,-1.82787223937844E-15,1.));
#29583=DIRECTION('ref_axis',(-1.,-3.04052209636688E-17,0.));
#29584=DIRECTION('',(0.382683432365093,-1.72396337974038E-15,0.923879532511285));
#29585=DIRECTION('center_axis',(0.,0.,-1.));
#29586=DIRECTION('ref_axis',(-1.,0.,0.));
#29587=DIRECTION('center_axis',(0.,0.,-1.));
#29588=DIRECTION('ref_axis',(-1.,0.,0.));
#29589=DIRECTION('center_axis',(0.,0.,1.));
#29590=DIRECTION('ref_axis',(1.,0.,0.));
#29591=DIRECTION('center_axis',(0.,0.,1.));
#29592=DIRECTION('ref_axis',(-1.,0.,0.));
#29593=DIRECTION('center_axis',(0.,0.,1.));
#29594=DIRECTION('ref_axis',(-1.,0.,0.));
#29595=DIRECTION('',(0.,0.,-1.));
#29596=DIRECTION('center_axis',(0.,-1.82787223937844E-15,-1.));
#29597=DIRECTION('ref_axis',(-1.,-3.04052209636688E-17,0.));
#29598=DIRECTION('center_axis',(0.,0.,-1.));
#29599=DIRECTION('ref_axis',(-1.,-6.12323399573677E-17,0.));
#29600=DIRECTION('',(0.382683432365093,-1.63023297163385E-15,-0.923879532511285));
#29601=DIRECTION('center_axis',(0.,0.,-1.));
#29602=DIRECTION('ref_axis',(-1.,0.,0.));
#29603=DIRECTION('center_axis',(0.,0.,1.));
#29604=DIRECTION('ref_axis',(-1.,-6.12323399573677E-17,0.));
#29605=DIRECTION('',(0.707106781186543,8.65956056235487E-17,-0.707106781186552));
#29606=DIRECTION('center_axis',(0.,0.,-1.));
#29607=DIRECTION('ref_axis',(-1.,0.,0.));
#29608=DIRECTION('center_axis',(0.,0.,-1.));
#29609=DIRECTION('ref_axis',(-1.,0.,0.));
#29610=DIRECTION('',(-0.707106781186555,8.65956056235503E-17,0.70710678118654));
#29611=DIRECTION('center_axis',(0.,0.,1.));
#29612=DIRECTION('ref_axis',(-1.,0.,0.));
#29613=DIRECTION('center_axis',(0.,0.,1.));
#29614=DIRECTION('ref_axis',(-1.,0.,0.));
#29615=DIRECTION('center_axis',(0.,0.,1.));
#29616=DIRECTION('ref_axis',(1.,0.,0.));
#29617=DIRECTION('center_axis',(0.,0.,-1.));
#29618=DIRECTION('ref_axis',(-1.,0.,0.));
#29619=DIRECTION('center_axis',(0.,0.,-1.));
#29620=DIRECTION('ref_axis',(-1.,0.,0.));
#29621=DIRECTION('',(0.,0.,-1.));
#29622=DIRECTION('center_axis',(0.,0.,-1.));
#29623=DIRECTION('ref_axis',(-1.,0.,0.));
#29624=DIRECTION('center_axis',(0.,4.39101262113477E-15,-1.));
#29625=DIRECTION('ref_axis',(-1.,-3.11403559978336E-17,0.));
#29626=DIRECTION('',(-0.923879532511284,-1.59599510772706E-15,0.382683432365097));
#29627=DIRECTION('center_axis',(0.,0.,-1.));
#29628=DIRECTION('ref_axis',(-1.,0.,0.));
#29629=DIRECTION('center_axis',(0.,0.,-1.));
#29630=DIRECTION('ref_axis',(-1.,0.,0.));
#29631=DIRECTION('center_axis',(0.,0.,-1.));
#29632=DIRECTION('ref_axis',(-1.,0.,0.));
#29633=DIRECTION('center_axis',(0.,0.,1.));
#29634=DIRECTION('ref_axis',(-1.,0.,0.));
#29635=DIRECTION('center_axis',(0.,0.,1.));
#29636=DIRECTION('ref_axis',(-1.,0.,0.));
#29637=DIRECTION('',(-0.707106781186555,-8.65956056235503E-17,-0.70710678118654));
#29638=DIRECTION('center_axis',(0.,0.,-1.));
#29639=DIRECTION('ref_axis',(-1.,0.,0.));
#29640=DIRECTION('center_axis',(0.,0.,-1.));
#29641=DIRECTION('ref_axis',(-1.,0.,0.));
#29642=DIRECTION('center_axis',(0.,0.,1.));
#29643=DIRECTION('ref_axis',(-1.,0.,0.));
#29644=DIRECTION('center_axis',(0.,0.,1.));
#29645=DIRECTION('ref_axis',(1.,0.,0.));
#29646=DIRECTION('center_axis',(0.,0.,1.));
#29647=DIRECTION('ref_axis',(1.,0.,0.));
#29648=DIRECTION('',(0.,0.,1.));
#29649=DIRECTION('center_axis',(0.,0.,1.));
#29650=DIRECTION('ref_axis',(-1.,0.,0.));
#29651=DIRECTION('center_axis',(0.,0.,1.));
#29652=DIRECTION('ref_axis',(-1.,0.,0.));
#29653=DIRECTION('',(-0.707106781186555,-8.65956056235503E-17,-0.70710678118654));
#29654=DIRECTION('center_axis',(0.,0.,-1.));
#29655=DIRECTION('ref_axis',(-1.,0.,0.));
#29656=DIRECTION('center_axis',(0.,0.,-1.));
#29657=DIRECTION('ref_axis',(-1.,0.,0.));
#29658=DIRECTION('center_axis',(0.,0.,1.));
#29659=DIRECTION('ref_axis',(-1.,0.,0.));
#29660=DIRECTION('center_axis',(0.,0.,1.));
#29661=DIRECTION('ref_axis',(1.,0.,0.));
#29662=DIRECTION('center_axis',(0.,0.,1.));
#29663=DIRECTION('ref_axis',(1.,0.,0.));
#29664=DIRECTION('',(0.,0.,1.));
#29665=DIRECTION('center_axis',(0.,0.,-1.));
#29666=DIRECTION('ref_axis',(1.,0.,0.));
#29667=DIRECTION('',(0.316227766016841,3.87267321454042E-17,0.948683298050513));
#29668=DIRECTION('center_axis',(0.,0.,1.));
#29669=DIRECTION('ref_axis',(1.,0.,0.));
#29670=DIRECTION('center_axis',(0.,0.,1.));
#29671=DIRECTION('ref_axis',(1.,0.,0.));
#29672=DIRECTION('',(0.,0.,1.));
#29673=DIRECTION('center_axis',(0.,0.,1.));
#29674=DIRECTION('ref_axis',(1.,0.,0.));
#29675=DIRECTION('center_axis',(0.,0.,1.));
#29676=DIRECTION('ref_axis',(1.,0.,0.));
#29677=DIRECTION('',(-0.707106781186542,-8.65956056235487E-17,0.707106781186553));
#29678=DIRECTION('center_axis',(0.,0.,1.));
#29679=DIRECTION('ref_axis',(1.,0.,0.));
#29680=DIRECTION('center_axis',(0.,0.,-1.));
#29681=DIRECTION('ref_axis',(-1.,0.,0.));
#29682=DIRECTION('center_axis',(0.,0.,-1.));
#29683=DIRECTION('ref_axis',(1.,0.,0.));
#29684=DIRECTION('',(0.316227766016841,3.87267321454042E-17,0.948683298050513));
#29685=DIRECTION('center_axis',(0.,0.,1.));
#29686=DIRECTION('ref_axis',(1.,0.,0.));
#29687=DIRECTION('center_axis',(0.,0.,1.));
#29688=DIRECTION('ref_axis',(1.,0.,0.));
#29689=DIRECTION('',(0.,0.,1.));
#29690=DIRECTION('center_axis',(0.,0.,1.));
#29691=DIRECTION('ref_axis',(1.,0.,0.));
#29692=DIRECTION('center_axis',(0.,0.,1.));
#29693=DIRECTION('ref_axis',(1.,0.,0.));
#29694=DIRECTION('',(-0.707106781186542,-8.65956056235487E-17,0.707106781186553));
#29695=DIRECTION('center_axis',(0.,0.,1.));
#29696=DIRECTION('ref_axis',(1.,0.,0.));
#29697=DIRECTION('center_axis',(0.,0.,-1.));
#29698=DIRECTION('ref_axis',(-1.,0.,0.));
#29699=DIRECTION('center_axis',(0.,0.,1.));
#29700=DIRECTION('ref_axis',(-1.,0.,0.));
#29701=DIRECTION('',(0.707106781186555,-8.65956056235503E-17,0.70710678118654));
#29702=DIRECTION('center_axis',(0.,0.,1.));
#29703=DIRECTION('ref_axis',(-1.,0.,0.));
#29704=DIRECTION('center_axis',(0.,0.,1.));
#29705=DIRECTION('ref_axis',(1.,0.,0.));
#35956=CARTESIAN_POINT('',(0.,0.,0.));
#35957=CARTESIAN_POINT('Origin',(0.,0.,12.615));
#35958=CARTESIAN_POINT('',(1.095,-1.34098824506635E-16,12.6));
#35959=CARTESIAN_POINT('Origin',(0.,0.,12.6));
#35960=CARTESIAN_POINT('',(1.065,1.30424884109193E-16,12.63));
#35961=CARTESIAN_POINT('',(1.08,-1.32261854307914E-16,12.615));
#35962=CARTESIAN_POINT('',(-1.065,-1.30424884109193E-16,12.63));
#35963=CARTESIAN_POINT('Origin',(0.,0.,12.63));
#35964=CARTESIAN_POINT('Origin',(0.,0.,12.63));
#35965=CARTESIAN_POINT('Origin',(1.55,0.,12.6));
#35966=CARTESIAN_POINT('',(1.47,1.80023079474661E-16,12.6));
#35967=CARTESIAN_POINT('Origin',(0.,0.,12.6));
#35968=CARTESIAN_POINT('',(-0.128333333333334,-1.28,12.6));
#35969=CARTESIAN_POINT('Origin',(0.,-1.28,12.6));
#35970=CARTESIAN_POINT('',(-0.128333333333334,1.28,12.6));
#35971=CARTESIAN_POINT('Origin',(0.,1.28,12.6));
#35972=CARTESIAN_POINT('Origin',(0.,0.,12.7));
#35973=CARTESIAN_POINT('',(-1.065,-1.30424884109193E-16,12.8));
#35974=CARTESIAN_POINT('Origin',(0.,0.,12.8));
#35975=CARTESIAN_POINT('',(-1.065,-1.30424884109193E-16,12.7));
#35976=CARTESIAN_POINT('Origin',(0.,4.65737220102024E-17,12.6106066017178));
#35977=CARTESIAN_POINT('',(1.5212132034356,0.,12.6212132034356));
#35978=CARTESIAN_POINT('Origin',(0.,9.31474440204048E-17,12.6212132034356));
#35979=CARTESIAN_POINT('',(1.4956066017178,2.7630642777814E-16,12.6106066017178));
#35980=CARTESIAN_POINT('Origin',(0.,0.,12.625));
#35981=CARTESIAN_POINT('',(1.5287867965644,3.74444771398267E-16,12.6287867965644));
#35982=CARTESIAN_POINT('Origin',(0.,9.36111928495666E-17,12.6287867965644));
#35983=CARTESIAN_POINT('',(1.525,1.86758636869971E-16,12.625));
#35984=CARTESIAN_POINT('Origin',(0.,4.68055964247833E-17,12.6543933982822));
#35985=CARTESIAN_POINT('',(1.55,-1.8982025386784E-16,12.68));
#35986=CARTESIAN_POINT('',(1.5393933982822,-9.49101269339199E-17,12.6543933982822));
#35987=CARTESIAN_POINT('',(-1.55,-1.8982025386784E-16,12.68));
#35988=CARTESIAN_POINT('Origin',(0.,0.,12.68));
#35989=CARTESIAN_POINT('Origin',(0.,0.,12.68));
#35990=CARTESIAN_POINT('Origin',(0.,0.,13.));
#35991=CARTESIAN_POINT('',(1.55,1.8982025386784E-16,13.32));
#35992=CARTESIAN_POINT('',(-1.55,-1.8982025386784E-16,13.32));
#35993=CARTESIAN_POINT('Origin',(0.,0.,13.32));
#35994=CARTESIAN_POINT('Origin',(0.,0.,13.32));
#35995=CARTESIAN_POINT('',(-1.55,-1.8982025386784E-16,13.));
#35996=CARTESIAN_POINT('Origin',(0.,4.68055964247833E-17,13.3456066017178));
#35997=CARTESIAN_POINT('',(1.5287867965644,0.,13.3712132034356));
#35998=CARTESIAN_POINT('Origin',(0.,9.36111928495666E-17,13.3712132034356));
#35999=CARTESIAN_POINT('',(1.5393933982822,2.82132512633053E-16,13.3456066017178));
#36000=CARTESIAN_POINT('Origin',(0.,0.,13.375));
#36001=CARTESIAN_POINT('',(1.5212132034356,3.72589776081619E-16,13.3787867965644));
#36002=CARTESIAN_POINT('Origin',(0.,9.31474440204048E-17,13.3787867965644));
#36003=CARTESIAN_POINT('',(1.525,1.86758636869971E-16,13.375));
#36004=CARTESIAN_POINT('Origin',(0.,0.,12.815));
#36005=CARTESIAN_POINT('',(0.94,-1.15116799119851E-16,12.8));
#36006=CARTESIAN_POINT('Origin',(0.,0.,12.8));
#36007=CARTESIAN_POINT('',(0.91,1.11442858722409E-16,12.83));
#36008=CARTESIAN_POINT('',(0.925,-1.1327982892113E-16,12.815));
#36009=CARTESIAN_POINT('',(-0.91,-1.11442858722409E-16,12.83));
#36010=CARTESIAN_POINT('Origin',(0.,0.,12.83));
#36011=CARTESIAN_POINT('Origin',(0.,0.,12.83));
#36012=CARTESIAN_POINT('Origin',(0.,0.,13.1));
#36013=CARTESIAN_POINT('',(0.91,-1.11442858722409E-16,13.36));
#36014=CARTESIAN_POINT('',(-0.91,-1.11442858722409E-16,13.36));
#36015=CARTESIAN_POINT('Origin',(0.,0.,13.36));
#36016=CARTESIAN_POINT('Origin',(0.,0.,13.36));
#36017=CARTESIAN_POINT('',(-0.91,-1.11442858722409E-16,13.1));
#36018=CARTESIAN_POINT('Origin',(1.065,0.,12.8));
#36019=CARTESIAN_POINT('Origin',(0.,4.65737220102024E-17,13.3893933982822));
#36020=CARTESIAN_POINT('',(1.46999999999999,-1.34246756157856E-16,13.4));
#36021=CARTESIAN_POINT('',(1.4956066017178,-9.00115397373305E-17,13.3893933982822));
#36022=CARTESIAN_POINT('',(0.156910396397301,-1.4616015625,13.4));
#36023=CARTESIAN_POINT('Origin',(0.,0.,13.4));
#36024=CARTESIAN_POINT('',(-0.156910396397301,-1.4616015625,13.4));
#36025=CARTESIAN_POINT('Ctrl Pts',(-0.156910396397299,-1.4616015625,13.4));
#36026=CARTESIAN_POINT('Ctrl Pts',(-0.149656402785207,-1.46593468366903,
13.3985361440069));
#36027=CARTESIAN_POINT('Ctrl Pts',(-0.142213279389795,-1.4699883651202,
13.3971707806262));
#36028=CARTESIAN_POINT('Ctrl Pts',(-0.0924978887707845,-1.49450064049362,
13.3889327354826));
#36029=CARTESIAN_POINT('Ctrl Pts',(-0.0452361545939354,-1.50535533905932,
13.3853553390593));
#36030=CARTESIAN_POINT('Ctrl Pts',(0.0452361545939354,-1.50535533905932,
13.3853553390593));
#36031=CARTESIAN_POINT('Ctrl Pts',(0.0924978887707845,-1.49450064049362,
13.3889327354826));
#36032=CARTESIAN_POINT('Ctrl Pts',(0.142213279389795,-1.4699883651202,13.3971707806262));
#36033=CARTESIAN_POINT('Ctrl Pts',(0.149656402785207,-1.46593468366903,
13.3985361440069));
#36034=CARTESIAN_POINT('Ctrl Pts',(0.156910396397299,-1.4616015625,13.4));
#36035=CARTESIAN_POINT('',(-0.156910396397301,1.4616015625,13.4));
#36036=CARTESIAN_POINT('Origin',(0.,0.,13.4));
#36037=CARTESIAN_POINT('',(0.156910396397301,1.4616015625,13.4));
#36038=CARTESIAN_POINT('Ctrl Pts',(0.156910396397303,1.4616015625,13.4));
#36039=CARTESIAN_POINT('Ctrl Pts',(0.149656402785211,1.46593468366904,13.3985361440069));
#36040=CARTESIAN_POINT('Ctrl Pts',(0.1422132793898,1.46998836512021,13.3971707806262));
#36041=CARTESIAN_POINT('Ctrl Pts',(0.0924978887707876,1.49450064049363,
13.3889327354826));
#36042=CARTESIAN_POINT('Ctrl Pts',(0.0452361545939373,1.50535533905933,
13.3853553390593));
#36043=CARTESIAN_POINT('Ctrl Pts',(-0.0452361545939372,1.50535533905933,
13.3853553390593));
#36044=CARTESIAN_POINT('Ctrl Pts',(-0.0924978887707876,1.49450064049363,
13.3889327354826));
#36045=CARTESIAN_POINT('Ctrl Pts',(-0.1422132793898,1.46998836512021,13.3971707806262));
#36046=CARTESIAN_POINT('Ctrl Pts',(-0.149656402785211,1.46593468366904,
13.3985361440069));
#36047=CARTESIAN_POINT('Ctrl Pts',(-0.156910396397303,1.4616015625,13.4));
#36048=CARTESIAN_POINT('Origin',(0.,0.,13.4));
#36049=CARTESIAN_POINT('Origin',(0.,1.28,13.385));
#36050=CARTESIAN_POINT('',(0.240000000000004,1.28,13.4));
#36051=CARTESIAN_POINT('Origin',(0.,1.28,13.4));
#36052=CARTESIAN_POINT('',(0.21,1.28,13.37));
#36053=CARTESIAN_POINT('',(0.225,1.28,13.385));
#36054=CARTESIAN_POINT('',(-0.21,1.28,13.37));
#36055=CARTESIAN_POINT('Origin',(0.,1.28,13.37));
#36056=CARTESIAN_POINT('Origin',(0.,1.28,13.37));
#36057=CARTESIAN_POINT('Origin',(0.,1.28,13.4));
#36058=CARTESIAN_POINT('Origin',(0.,1.28,13.29));
#36059=CARTESIAN_POINT('',(-0.21,1.28,13.18));
#36060=CARTESIAN_POINT('Origin',(0.,1.28,13.18));
#36061=CARTESIAN_POINT('',(-0.21,1.28,13.29));
#36062=CARTESIAN_POINT('Origin',(0.,-1.28,13.385));
#36063=CARTESIAN_POINT('',(0.24,-1.28,13.4));
#36064=CARTESIAN_POINT('Origin',(0.,-1.28,13.4));
#36065=CARTESIAN_POINT('',(0.21,-1.28,13.37));
#36066=CARTESIAN_POINT('',(0.225,-1.28,13.385));
#36067=CARTESIAN_POINT('',(-0.21,-1.28,13.37));
#36068=CARTESIAN_POINT('Origin',(0.,-1.28,13.37));
#36069=CARTESIAN_POINT('Origin',(0.,-1.28,13.37));
#36070=CARTESIAN_POINT('Origin',(0.,-1.28,13.4));
#36071=CARTESIAN_POINT('Origin',(0.,-1.28,13.29));
#36072=CARTESIAN_POINT('',(-0.21,-1.28,13.18));
#36073=CARTESIAN_POINT('Origin',(0.,-1.28,13.18));
#36074=CARTESIAN_POINT('',(-0.21,-1.28,13.29));
#36075=CARTESIAN_POINT('Origin',(0.,-1.28,12.5875));
#36076=CARTESIAN_POINT('',(-0.12,-1.28,12.625));
#36077=CARTESIAN_POINT('',(-0.1325,-1.28,12.5875));
#36078=CARTESIAN_POINT('Origin',(0.,-1.28,12.625));
#36079=CARTESIAN_POINT('Origin',(0.,-1.28,12.89));
#36080=CARTESIAN_POINT('',(-0.12,-1.28,13.155));
#36081=CARTESIAN_POINT('',(-0.12,-1.28,12.89));
#36082=CARTESIAN_POINT('Origin',(0.,-1.28,13.155));
#36083=CARTESIAN_POINT('Origin',(0.,-1.28,13.1675));
#36084=CARTESIAN_POINT('',(-0.145,-1.28,13.18));
#36085=CARTESIAN_POINT('',(-0.1325,-1.28,13.1675));
#36086=CARTESIAN_POINT('Origin',(0.,-1.28,13.18));
#36087=CARTESIAN_POINT('Origin',(0.21,-1.28,13.18));
#36088=CARTESIAN_POINT('Origin',(0.,1.28,12.5875));
#36089=CARTESIAN_POINT('',(-0.12,1.28,12.625));
#36090=CARTESIAN_POINT('',(-0.1325,1.28,12.5875));
#36091=CARTESIAN_POINT('Origin',(0.,1.28,12.625));
#36092=CARTESIAN_POINT('Origin',(0.,1.28,12.89));
#36093=CARTESIAN_POINT('',(-0.12,1.28,13.155));
#36094=CARTESIAN_POINT('',(-0.12,1.28,12.89));
#36095=CARTESIAN_POINT('Origin',(0.,1.28,13.155));
#36096=CARTESIAN_POINT('Origin',(0.,1.28,13.1675));
#36097=CARTESIAN_POINT('',(-0.145,1.28,13.18));
#36098=CARTESIAN_POINT('',(-0.1325,1.28,13.1675));
#36099=CARTESIAN_POINT('Origin',(0.,1.28,13.18));
#36100=CARTESIAN_POINT('Origin',(0.21,1.28,13.18));
#36101=CARTESIAN_POINT('Origin',(0.,0.,13.38));
#36102=CARTESIAN_POINT('',(0.95,1.16341445918999E-16,13.4));
#36103=CARTESIAN_POINT('',(0.93,-1.13892152320704E-16,13.38));
#36104=CARTESIAN_POINT('Origin',(0.,0.,13.4));
#36105=CARTESIAN_POINT('Origin',(0.91,0.,13.4));
#54964=UNCERTAINTY_MEASURE_WITH_UNIT(LENGTH_MEASURE(0.001),#55003,
'DISTANCE_ACCURACY_VALUE',
'Maximum model space distance between geometric entities at asserted c
onnectivities');
#54980=UNCERTAINTY_MEASURE_WITH_UNIT(LENGTH_MEASURE(0.001),#55003,
'DISTANCE_ACCURACY_VALUE',
'Maximum model space distance between geometric entities at asserted c
onnectivities');
#54986=(
GEOMETRIC_REPRESENTATION_CONTEXT(3)
GLOBAL_UNCERTAINTY_ASSIGNED_CONTEXT((#54964))
GLOBAL_UNIT_ASSIGNED_CONTEXT((#55003,#55005,#55006))
REPRESENTATION_CONTEXT('','3D')
);
#55002=(
GEOMETRIC_REPRESENTATION_CONTEXT(3)
GLOBAL_UNCERTAINTY_ASSIGNED_CONTEXT((#54980))
GLOBAL_UNIT_ASSIGNED_CONTEXT((#55003,#55005,#55006))
REPRESENTATION_CONTEXT('','3D')
);
#55003=(
LENGTH_UNIT()
NAMED_UNIT(*)
SI_UNIT(.CENTI.,.METRE.)
);
#55005=(
NAMED_UNIT(*)
PLANE_ANGLE_UNIT()
SI_UNIT($,.RADIAN.)
);
#55006=(
NAMED_UNIT(*)
SI_UNIT($,.STERADIAN.)
SOLID_ANGLE_UNIT()
);
#55012=SHAPE_DEFINITION_REPRESENTATION(#55033,#55108);
#55033=PRODUCT_DEFINITION_SHAPE('',$,#55130);
#55108=SHAPE_REPRESENTATION('',(#25681),#54986);
#55124=PRODUCT_DEFINITION_CONTEXT('part definition',#55189,'design');
#55130=PRODUCT_DEFINITION('2026-10-18-23-36-10-777',
'05_Port_Clamp_Collar_D31',#55151,#55124);
#55151=PRODUCT_DEFINITION_FORMATION('',$,#55196);
#55189=APPLICATION_CONTEXT(
'Core Data for Automotive Mechanical Design Process');
#55190=PRODUCT_CONTEXT('part definition',#55189,'mechanical');
#55196=PRODUCT('2026-10-18-23-36-10-777','05_Port_Clamp_Collar_D31',$,(#55190));
#55373=COLOUR_RGB('Sky Blue',0.24,0.69,0.87);
#55374=FILL_AREA_STYLE_COLOUR('',#55373);
#55375=FILL_AREA_STYLE('',(#55374));
#55376=SURFACE_STYLE_FILL_AREA(#55375);
#55377=SURFACE_SIDE_STYLE('',(#55376));
#55378=SURFACE_STYLE_USAGE(.BOTH.,#55377);
#55379=PRESENTATION_STYLE_ASSIGNMENT((#55378));
ENDSEC;
END-ISO-10303-21;
